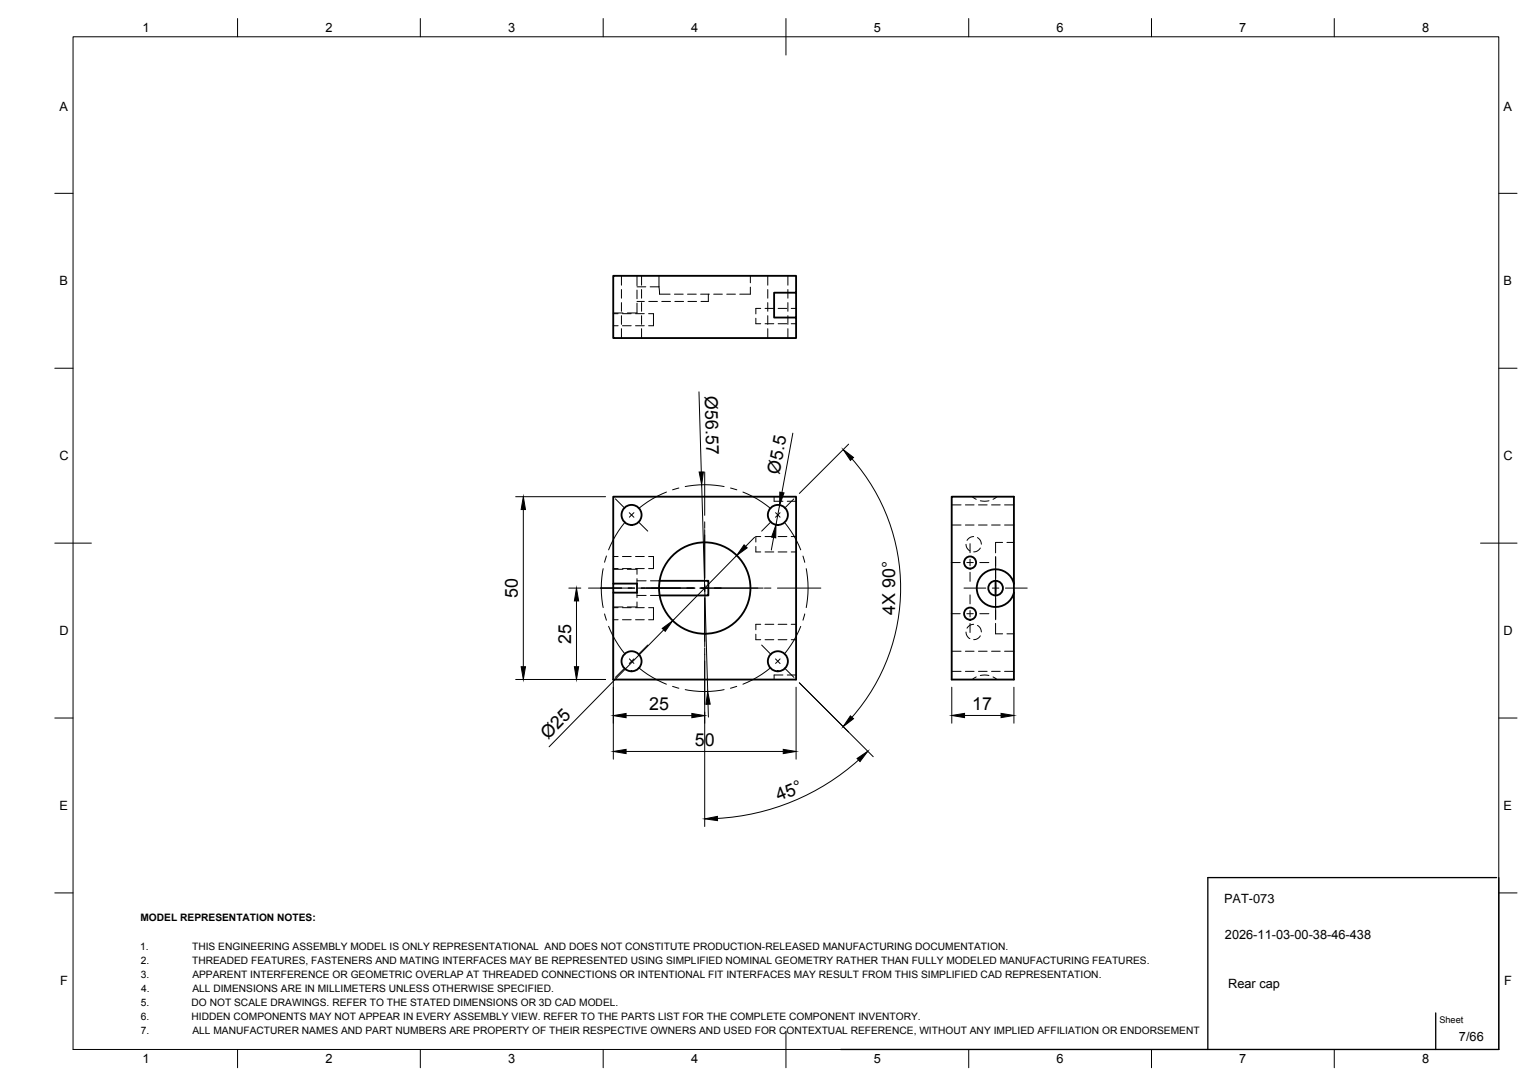
ISO-10303-21;
HEADER;
/* Generated by software containing ST-Developer
 * from STEP Tools, Inc. (www.steptools.com) 
 */

FILE_DESCRIPTION(
/* description */ ('Manual piston pump'),
/* implementation_level */ '2;1');

FILE_NAME(
/* name */ 'Rear cap.step',
/* time_stamp */ '2026-11-02T16:54:23-08:00',
/* author */ (''),
/* organization */ (''),
/* preprocessor_version */ 'ST-DEVELOPER v20.2',
/* originating_system */ 'Autodesk Translation Framework v15.17.0.0',
/* authorisation */ '');

FILE_SCHEMA (('AUTOMOTIVE_DESIGN { 1 0 10303 214 3 1 1 }'));
ENDSEC;

DATA;
#10=MECHANICAL_DESIGN_GEOMETRIC_PRESENTATION_REPRESENTATION('',(#690),#19043);
#564=SHAPE_REPRESENTATION_RELATIONSHIP('SRR','None',#19310,#627);
#627=ADVANCED_BREP_SHAPE_REPRESENTATION('',(#762),#18977);
#690=STYLED_ITEM('',(#19661),#762);
#762=MANIFOLD_SOLID_BREP('Body1',#9474);
#850=FACE_BOUND('',#1945,.T.);
#851=FACE_BOUND('',#1948,.T.);
#852=FACE_BOUND('',#1949,.T.);
#853=FACE_BOUND('',#1950,.T.);
#854=FACE_BOUND('',#1951,.T.);
#855=FACE_BOUND('',#1952,.T.);
#856=FACE_BOUND('',#1959,.T.);
#857=FACE_BOUND('',#1960,.T.);
#858=FACE_BOUND('',#1961,.T.);
#859=FACE_BOUND('',#1962,.T.);
#860=FACE_BOUND('',#1965,.T.);
#861=FACE_BOUND('',#1966,.T.);
#862=FACE_BOUND('',#1968,.T.);
#863=FACE_BOUND('',#1969,.T.);
#1050=B_SPLINE_CURVE_WITH_KNOTS('',3,(#14902,#14903,#14904,#14905,#14906,
#14907,#14908,#14909,#14910,#14911,#14912,#14913,#14914,#14915,#14916,#14917,
#14918,#14919),.UNSPECIFIED.,.F.,.F.,(4,2,2,2,2,2,2,2,4),(-0.603815071984235,
-0.528337333647547,-0.45285959531086,-0.377383565651489,-0.301907535992118,
-0.226431506332746,-0.150955476673375,-0.0754777383366876,0.),
 .UNSPECIFIED.);
#1109=CYLINDRICAL_SURFACE('',#10323,0.165);
#1110=CYLINDRICAL_SURFACE('',#10327,0.165);
#1111=CYLINDRICAL_SURFACE('',#10333,0.525);
#1112=CYLINDRICAL_SURFACE('',#10335,0.525);
#1113=CYLINDRICAL_SURFACE('',#10340,0.21);
#1114=CYLINDRICAL_SURFACE('',#10344,0.21);
#1115=CYLINDRICAL_SURFACE('',#10350,0.2);
#1116=CYLINDRICAL_SURFACE('',#10357,0.515);
#1117=CYLINDRICAL_SURFACE('',#10365,0.275);
#1118=CYLINDRICAL_SURFACE('',#10367,0.275);
#1119=CYLINDRICAL_SURFACE('',#10369,0.275);
#1120=CYLINDRICAL_SURFACE('',#10371,0.275);
#1121=CYLINDRICAL_SURFACE('',#10373,1.25);
#1330=FACE_OUTER_BOUND('',#1928,.T.);
#1331=FACE_OUTER_BOUND('',#1929,.T.);
#1332=FACE_OUTER_BOUND('',#1930,.T.);
#1333=FACE_OUTER_BOUND('',#1931,.T.);
#1334=FACE_OUTER_BOUND('',#1932,.T.);
#1335=FACE_OUTER_BOUND('',#1933,.T.);
#1336=FACE_OUTER_BOUND('',#1934,.T.);
#1337=FACE_OUTER_BOUND('',#1935,.T.);
#1338=FACE_OUTER_BOUND('',#1936,.T.);
#1339=FACE_OUTER_BOUND('',#1937,.T.);
#1340=FACE_OUTER_BOUND('',#1938,.T.);
#1341=FACE_OUTER_BOUND('',#1939,.T.);
#1342=FACE_OUTER_BOUND('',#1940,.T.);
#1343=FACE_OUTER_BOUND('',#1941,.T.);
#1344=FACE_OUTER_BOUND('',#1942,.T.);
#1345=FACE_OUTER_BOUND('',#1943,.T.);
#1346=FACE_OUTER_BOUND('',#1944,.T.);
#1347=FACE_OUTER_BOUND('',#1946,.T.);
#1348=FACE_OUTER_BOUND('',#1947,.T.);
#1349=FACE_OUTER_BOUND('',#1953,.T.);
#1350=FACE_OUTER_BOUND('',#1954,.T.);
#1351=FACE_OUTER_BOUND('',#1955,.T.);
#1352=FACE_OUTER_BOUND('',#1956,.T.);
#1353=FACE_OUTER_BOUND('',#1957,.T.);
#1354=FACE_OUTER_BOUND('',#1958,.T.);
#1355=FACE_OUTER_BOUND('',#1963,.T.);
#1356=FACE_OUTER_BOUND('',#1964,.T.);
#1357=FACE_OUTER_BOUND('',#1967,.T.);
#1928=EDGE_LOOP('',(#6457,#6458,#6459,#6460));
#1929=EDGE_LOOP('',(#6461));
#1930=EDGE_LOOP('',(#6462,#6463,#6464,#6465));
#1931=EDGE_LOOP('',(#6466));
#1932=EDGE_LOOP('',(#6467,#6468));
#1933=EDGE_LOOP('',(#6469,#6470,#6471,#6472));
#1934=EDGE_LOOP('',(#6473,#6474,#6475,#6476));
#1935=EDGE_LOOP('',(#6477,#6478));
#1936=EDGE_LOOP('',(#6479,#6480,#6481,#6482,#6483,#6484,#6485,#6486));
#1937=EDGE_LOOP('',(#6487,#6488,#6489,#6490));
#1938=EDGE_LOOP('',(#6491));
#1939=EDGE_LOOP('',(#6492,#6493,#6494,#6495));
#1940=EDGE_LOOP('',(#6496));
#1941=EDGE_LOOP('',(#6497,#6498));
#1942=EDGE_LOOP('',(#6499,#6500,#6501,#6502,#6503,#6504,#6505));
#1943=EDGE_LOOP('',(#6506,#6507,#6508,#6509,#6510));
#1944=EDGE_LOOP('',(#6511,#6512));
#1945=EDGE_LOOP('',(#6513));
#1946=EDGE_LOOP('',(#6514,#6515,#6516,#6517));
#1947=EDGE_LOOP('',(#6518,#6519,#6520,#6521,#6522,#6523,#6524,#6525));
#1948=EDGE_LOOP('',(#6526));
#1949=EDGE_LOOP('',(#6527));
#1950=EDGE_LOOP('',(#6528));
#1951=EDGE_LOOP('',(#6529));
#1952=EDGE_LOOP('',(#6530));
#1953=EDGE_LOOP('',(#6531,#6532,#6533,#6534));
#1954=EDGE_LOOP('',(#6535,#6536,#6537,#6538));
#1955=EDGE_LOOP('',(#6539,#6540,#6541,#6542));
#1956=EDGE_LOOP('',(#6543,#6544,#6545,#6546));
#1957=EDGE_LOOP('',(#6547,#6548,#6549,#6550,#6551,#6552));
#1958=EDGE_LOOP('',(#6553,#6554,#6555,#6556));
#1959=EDGE_LOOP('',(#6557));
#1960=EDGE_LOOP('',(#6558));
#1961=EDGE_LOOP('',(#6559));
#1962=EDGE_LOOP('',(#6560));
#1963=EDGE_LOOP('',(#6561,#6562,#6563,#6564,#6565,#6566,#6567,#6568));
#1964=EDGE_LOOP('',(#6569,#6570,#6571,#6572,#6573,#6574));
#1965=EDGE_LOOP('',(#6575));
#1966=EDGE_LOOP('',(#6576));
#1967=EDGE_LOOP('',(#6577,#6578,#6579,#6580,#6581,#6582,#6583,#6584));
#1968=EDGE_LOOP('',(#6585));
#1969=EDGE_LOOP('',(#6586));
#2700=CIRCLE('',#10324,0.165);
#2701=CIRCLE('',#10325,0.165);
#2702=CIRCLE('',#10328,0.165);
#2703=CIRCLE('',#10329,0.165);
#2704=CIRCLE('',#10332,0.525);
#2705=CIRCLE('',#10334,0.525);
#2706=CIRCLE('',#10336,0.525);
#2707=CIRCLE('',#10337,0.525);
#2708=CIRCLE('',#10341,0.21);
#2709=CIRCLE('',#10342,0.21);
#2710=CIRCLE('',#10345,0.21);
#2711=CIRCLE('',#10346,0.21);
#2712=CIRCLE('',#10349,0.2);
#2713=CIRCLE('',#10351,0.2);
#2714=CIRCLE('',#10353,1.25);
#2715=CIRCLE('',#10354,1.25);
#2716=CIRCLE('',#10356,0.515);
#2717=CIRCLE('',#10358,0.515);
#2718=CIRCLE('',#10360,0.275);
#2719=CIRCLE('',#10361,0.275);
#2720=CIRCLE('',#10362,0.275);
#2721=CIRCLE('',#10363,0.275);
#2722=CIRCLE('',#10364,1.25);
#2723=CIRCLE('',#10366,0.275);
#2724=CIRCLE('',#10368,0.275);
#2725=CIRCLE('',#10370,0.275);
#2726=CIRCLE('',#10372,0.275);
#3200=LINE('',#14837,#3804);
#3201=LINE('',#14844,#3805);
#3202=LINE('',#14850,#3806);
#3203=LINE('',#14854,#3807);
#3204=LINE('',#14857,#3808);
#3205=LINE('',#14861,#3809);
#3206=LINE('',#14865,#3810);
#3207=LINE('',#14868,#3811);
#3208=LINE('',#14871,#3812);
#3209=LINE('',#14873,#3813);
#3210=LINE('',#14875,#3814);
#3211=LINE('',#14877,#3815);
#3212=LINE('',#14878,#3816);
#3213=LINE('',#14883,#3817);
#3214=LINE('',#14890,#3818);
#3215=LINE('',#14896,#3819);
#3216=LINE('',#14900,#3820);
#3217=LINE('',#14921,#3821);
#3218=LINE('',#14923,#3822);
#3219=LINE('',#14931,#3823);
#3220=LINE('',#14935,#3824);
#3221=LINE('',#14938,#3825);
#3222=LINE('',#14940,#3826);
#3223=LINE('',#14942,#3827);
#3224=LINE('',#14944,#3828);
#3225=LINE('',#14945,#3829);
#3226=LINE('',#14958,#3830);
#3227=LINE('',#14962,#3831);
#3228=LINE('',#14966,#3832);
#3229=LINE('',#14970,#3833);
#3230=LINE('',#14973,#3834);
#3231=LINE('',#14976,#3835);
#3232=LINE('',#14978,#3836);
#3233=LINE('',#14979,#3837);
#3234=LINE('',#14981,#3838);
#3235=LINE('',#14982,#3839);
#3236=LINE('',#14983,#3840);
#3804=VECTOR('',#11712,0.165);
#3805=VECTOR('',#11721,0.165);
#3806=VECTOR('',#11728,1.);
#3807=VECTOR('',#11733,1.);
#3808=VECTOR('',#11736,1.);
#3809=VECTOR('',#11739,1.);
#3810=VECTOR('',#11742,1.);
#3811=VECTOR('',#11747,1.);
#3812=VECTOR('',#11750,1.);
#3813=VECTOR('',#11751,1.);
#3814=VECTOR('',#11752,1.);
#3815=VECTOR('',#11753,1.);
#3816=VECTOR('',#11754,1.);
#3817=VECTOR('',#11759,0.21);
#3818=VECTOR('',#11768,0.21);
#3819=VECTOR('',#11775,1.);
#3820=VECTOR('',#11780,1.);
#3821=VECTOR('',#11781,0.2);
#3822=VECTOR('',#11784,1.);
#3823=VECTOR('',#11793,1.);
#3824=VECTOR('',#11798,1.);
#3825=VECTOR('',#11801,1.);
#3826=VECTOR('',#11804,1.);
#3827=VECTOR('',#11805,1.);
#3828=VECTOR('',#11806,1.);
#3829=VECTOR('',#11807,1.);
#3830=VECTOR('',#11820,0.275);
#3831=VECTOR('',#11825,0.275);
#3832=VECTOR('',#11830,0.275);
#3833=VECTOR('',#11835,0.275);
#3834=VECTOR('',#11840,1.25);
#3835=VECTOR('',#11843,1.);
#3836=VECTOR('',#11844,1.);
#3837=VECTOR('',#11845,1.);
#3838=VECTOR('',#11848,1.);
#3839=VECTOR('',#11849,1.);
#3840=VECTOR('',#11850,1.);
#4416=VERTEX_POINT('',#14834);
#4417=VERTEX_POINT('',#14836);
#4418=VERTEX_POINT('',#14841);
#4419=VERTEX_POINT('',#14843);
#4420=VERTEX_POINT('',#14848);
#4421=VERTEX_POINT('',#14849);
#4422=VERTEX_POINT('',#14853);
#4423=VERTEX_POINT('',#14855);
#4424=VERTEX_POINT('',#14859);
#4425=VERTEX_POINT('',#14860);
#4426=VERTEX_POINT('',#14862);
#4427=VERTEX_POINT('',#14864);
#4428=VERTEX_POINT('',#14870);
#4429=VERTEX_POINT('',#14872);
#4430=VERTEX_POINT('',#14874);
#4431=VERTEX_POINT('',#14876);
#4432=VERTEX_POINT('',#14880);
#4433=VERTEX_POINT('',#14882);
#4434=VERTEX_POINT('',#14887);
#4435=VERTEX_POINT('',#14889);
#4436=VERTEX_POINT('',#14894);
#4437=VERTEX_POINT('',#14895);
#4438=VERTEX_POINT('',#14899);
#4439=VERTEX_POINT('',#14901);
#4440=VERTEX_POINT('',#14920);
#4441=VERTEX_POINT('',#14925);
#4442=VERTEX_POINT('',#14929);
#4443=VERTEX_POINT('',#14930);
#4444=VERTEX_POINT('',#14934);
#4445=VERTEX_POINT('',#14936);
#4446=VERTEX_POINT('',#14941);
#4447=VERTEX_POINT('',#14943);
#4448=VERTEX_POINT('',#14946);
#4449=VERTEX_POINT('',#14948);
#4450=VERTEX_POINT('',#14950);
#4451=VERTEX_POINT('',#14952);
#4452=VERTEX_POINT('',#14954);
#4453=VERTEX_POINT('',#14957);
#4454=VERTEX_POINT('',#14961);
#4455=VERTEX_POINT('',#14965);
#4456=VERTEX_POINT('',#14969);
#4457=VERTEX_POINT('',#14975);
#4458=VERTEX_POINT('',#14977);
#5215=EDGE_CURVE('',#4416,#4416,#2700,.T.);
#5216=EDGE_CURVE('',#4416,#4417,#3200,.T.);
#5217=EDGE_CURVE('',#4417,#4417,#2701,.T.);
#5218=EDGE_CURVE('',#4418,#4418,#2702,.T.);
#5219=EDGE_CURVE('',#4418,#4419,#3201,.T.);
#5220=EDGE_CURVE('',#4419,#4419,#2703,.T.);
#5221=EDGE_CURVE('',#4420,#4421,#3202,.T.);
#5222=EDGE_CURVE('',#4421,#4420,#2704,.T.);
#5223=EDGE_CURVE('',#4422,#4420,#3203,.T.);
#5224=EDGE_CURVE('',#4423,#4422,#2705,.T.);
#5225=EDGE_CURVE('',#4421,#4423,#3204,.T.);
#5226=EDGE_CURVE('',#4424,#4425,#3205,.T.);
#5227=EDGE_CURVE('',#4424,#4426,#2706,.T.);
#5228=EDGE_CURVE('',#4427,#4426,#3206,.T.);
#5229=EDGE_CURVE('',#4425,#4427,#2707,.T.);
#5230=EDGE_CURVE('',#4426,#4424,#3207,.T.);
#5231=EDGE_CURVE('',#4423,#4428,#3208,.T.);
#5232=EDGE_CURVE('',#4428,#4429,#3209,.T.);
#5233=EDGE_CURVE('',#4430,#4429,#3210,.T.);
#5234=EDGE_CURVE('',#4431,#4430,#3211,.T.);
#5235=EDGE_CURVE('',#4431,#4422,#3212,.T.);
#5236=EDGE_CURVE('',#4432,#4432,#2708,.T.);
#5237=EDGE_CURVE('',#4432,#4433,#3213,.T.);
#5238=EDGE_CURVE('',#4433,#4433,#2709,.T.);
#5239=EDGE_CURVE('',#4434,#4434,#2710,.T.);
#5240=EDGE_CURVE('',#4434,#4435,#3214,.T.);
#5241=EDGE_CURVE('',#4435,#4435,#2711,.T.);
#5242=EDGE_CURVE('',#4436,#4437,#3215,.T.);
#5243=EDGE_CURVE('',#4436,#4437,#2712,.T.);
#5244=EDGE_CURVE('',#4438,#4436,#3216,.T.);
#5245=EDGE_CURVE('',#4439,#4438,#1050,.T.);
#5246=EDGE_CURVE('',#4439,#4440,#3217,.T.);
#5247=EDGE_CURVE('',#4440,#4440,#2713,.T.);
#5248=EDGE_CURVE('',#4437,#4439,#3218,.T.);
#5249=EDGE_CURVE('',#4441,#4439,#2714,.T.);
#5250=EDGE_CURVE('',#4438,#4441,#2715,.T.);
#5251=EDGE_CURVE('',#4442,#4443,#3219,.T.);
#5252=EDGE_CURVE('',#4442,#4443,#2716,.T.);
#5253=EDGE_CURVE('',#4444,#4442,#3220,.T.);
#5254=EDGE_CURVE('',#4445,#4444,#2717,.T.);
#5255=EDGE_CURVE('',#4443,#4445,#3221,.T.);
#5256=EDGE_CURVE('',#4429,#4445,#3222,.T.);
#5257=EDGE_CURVE('',#4428,#4446,#3223,.T.);
#5258=EDGE_CURVE('',#4446,#4447,#3224,.T.);
#5259=EDGE_CURVE('',#4444,#4447,#3225,.T.);
#5260=EDGE_CURVE('',#4448,#4448,#2718,.T.);
#5261=EDGE_CURVE('',#4449,#4449,#2719,.T.);
#5262=EDGE_CURVE('',#4450,#4450,#2720,.T.);
#5263=EDGE_CURVE('',#4451,#4451,#2721,.T.);
#5264=EDGE_CURVE('',#4452,#4452,#2722,.T.);
#5265=EDGE_CURVE('',#4448,#4453,#3226,.T.);
#5266=EDGE_CURVE('',#4453,#4453,#2723,.T.);
#5267=EDGE_CURVE('',#4449,#4454,#3227,.T.);
#5268=EDGE_CURVE('',#4454,#4454,#2724,.T.);
#5269=EDGE_CURVE('',#4450,#4455,#3228,.T.);
#5270=EDGE_CURVE('',#4455,#4455,#2725,.T.);
#5271=EDGE_CURVE('',#4451,#4456,#3229,.T.);
#5272=EDGE_CURVE('',#4456,#4456,#2726,.T.);
#5273=EDGE_CURVE('',#4452,#4441,#3230,.T.);
#5274=EDGE_CURVE('',#4457,#4431,#3231,.T.);
#5275=EDGE_CURVE('',#4458,#4430,#3232,.T.);
#5276=EDGE_CURVE('',#4457,#4458,#3233,.T.);
#5277=EDGE_CURVE('',#4425,#4457,#3234,.T.);
#5278=EDGE_CURVE('',#4447,#4458,#3235,.T.);
#5279=EDGE_CURVE('',#4446,#4427,#3236,.T.);
#6457=ORIENTED_EDGE('',*,*,#5215,.F.);
#6458=ORIENTED_EDGE('',*,*,#5216,.T.);
#6459=ORIENTED_EDGE('',*,*,#5217,.F.);
#6460=ORIENTED_EDGE('',*,*,#5216,.F.);
#6461=ORIENTED_EDGE('',*,*,#5215,.T.);
#6462=ORIENTED_EDGE('',*,*,#5218,.F.);
#6463=ORIENTED_EDGE('',*,*,#5219,.T.);
#6464=ORIENTED_EDGE('',*,*,#5220,.F.);
#6465=ORIENTED_EDGE('',*,*,#5219,.F.);
#6466=ORIENTED_EDGE('',*,*,#5218,.T.);
#6467=ORIENTED_EDGE('',*,*,#5221,.F.);
#6468=ORIENTED_EDGE('',*,*,#5222,.F.);
#6469=ORIENTED_EDGE('',*,*,#5223,.F.);
#6470=ORIENTED_EDGE('',*,*,#5224,.F.);
#6471=ORIENTED_EDGE('',*,*,#5225,.F.);
#6472=ORIENTED_EDGE('',*,*,#5222,.T.);
#6473=ORIENTED_EDGE('',*,*,#5226,.F.);
#6474=ORIENTED_EDGE('',*,*,#5227,.T.);
#6475=ORIENTED_EDGE('',*,*,#5228,.F.);
#6476=ORIENTED_EDGE('',*,*,#5229,.F.);
#6477=ORIENTED_EDGE('',*,*,#5230,.F.);
#6478=ORIENTED_EDGE('',*,*,#5227,.F.);
#6479=ORIENTED_EDGE('',*,*,#5223,.T.);
#6480=ORIENTED_EDGE('',*,*,#5221,.T.);
#6481=ORIENTED_EDGE('',*,*,#5225,.T.);
#6482=ORIENTED_EDGE('',*,*,#5231,.T.);
#6483=ORIENTED_EDGE('',*,*,#5232,.T.);
#6484=ORIENTED_EDGE('',*,*,#5233,.F.);
#6485=ORIENTED_EDGE('',*,*,#5234,.F.);
#6486=ORIENTED_EDGE('',*,*,#5235,.T.);
#6487=ORIENTED_EDGE('',*,*,#5236,.F.);
#6488=ORIENTED_EDGE('',*,*,#5237,.T.);
#6489=ORIENTED_EDGE('',*,*,#5238,.T.);
#6490=ORIENTED_EDGE('',*,*,#5237,.F.);
#6491=ORIENTED_EDGE('',*,*,#5238,.F.);
#6492=ORIENTED_EDGE('',*,*,#5239,.F.);
#6493=ORIENTED_EDGE('',*,*,#5240,.T.);
#6494=ORIENTED_EDGE('',*,*,#5241,.T.);
#6495=ORIENTED_EDGE('',*,*,#5240,.F.);
#6496=ORIENTED_EDGE('',*,*,#5241,.F.);
#6497=ORIENTED_EDGE('',*,*,#5242,.F.);
#6498=ORIENTED_EDGE('',*,*,#5243,.T.);
#6499=ORIENTED_EDGE('',*,*,#5244,.F.);
#6500=ORIENTED_EDGE('',*,*,#5245,.F.);
#6501=ORIENTED_EDGE('',*,*,#5246,.T.);
#6502=ORIENTED_EDGE('',*,*,#5247,.F.);
#6503=ORIENTED_EDGE('',*,*,#5246,.F.);
#6504=ORIENTED_EDGE('',*,*,#5248,.F.);
#6505=ORIENTED_EDGE('',*,*,#5243,.F.);
#6506=ORIENTED_EDGE('',*,*,#5244,.T.);
#6507=ORIENTED_EDGE('',*,*,#5242,.T.);
#6508=ORIENTED_EDGE('',*,*,#5248,.T.);
#6509=ORIENTED_EDGE('',*,*,#5249,.F.);
#6510=ORIENTED_EDGE('',*,*,#5250,.F.);
#6511=ORIENTED_EDGE('',*,*,#5251,.F.);
#6512=ORIENTED_EDGE('',*,*,#5252,.T.);
#6513=ORIENTED_EDGE('',*,*,#5247,.T.);
#6514=ORIENTED_EDGE('',*,*,#5253,.F.);
#6515=ORIENTED_EDGE('',*,*,#5254,.F.);
#6516=ORIENTED_EDGE('',*,*,#5255,.F.);
#6517=ORIENTED_EDGE('',*,*,#5252,.F.);
#6518=ORIENTED_EDGE('',*,*,#5253,.T.);
#6519=ORIENTED_EDGE('',*,*,#5251,.T.);
#6520=ORIENTED_EDGE('',*,*,#5255,.T.);
#6521=ORIENTED_EDGE('',*,*,#5256,.F.);
#6522=ORIENTED_EDGE('',*,*,#5232,.F.);
#6523=ORIENTED_EDGE('',*,*,#5257,.T.);
#6524=ORIENTED_EDGE('',*,*,#5258,.T.);
#6525=ORIENTED_EDGE('',*,*,#5259,.F.);
#6526=ORIENTED_EDGE('',*,*,#5260,.T.);
#6527=ORIENTED_EDGE('',*,*,#5261,.T.);
#6528=ORIENTED_EDGE('',*,*,#5262,.T.);
#6529=ORIENTED_EDGE('',*,*,#5263,.T.);
#6530=ORIENTED_EDGE('',*,*,#5264,.T.);
#6531=ORIENTED_EDGE('',*,*,#5260,.F.);
#6532=ORIENTED_EDGE('',*,*,#5265,.T.);
#6533=ORIENTED_EDGE('',*,*,#5266,.F.);
#6534=ORIENTED_EDGE('',*,*,#5265,.F.);
#6535=ORIENTED_EDGE('',*,*,#5261,.F.);
#6536=ORIENTED_EDGE('',*,*,#5267,.T.);
#6537=ORIENTED_EDGE('',*,*,#5268,.F.);
#6538=ORIENTED_EDGE('',*,*,#5267,.F.);
#6539=ORIENTED_EDGE('',*,*,#5262,.F.);
#6540=ORIENTED_EDGE('',*,*,#5269,.T.);
#6541=ORIENTED_EDGE('',*,*,#5270,.F.);
#6542=ORIENTED_EDGE('',*,*,#5269,.F.);
#6543=ORIENTED_EDGE('',*,*,#5263,.F.);
#6544=ORIENTED_EDGE('',*,*,#5271,.T.);
#6545=ORIENTED_EDGE('',*,*,#5272,.F.);
#6546=ORIENTED_EDGE('',*,*,#5271,.F.);
#6547=ORIENTED_EDGE('',*,*,#5264,.F.);
#6548=ORIENTED_EDGE('',*,*,#5273,.T.);
#6549=ORIENTED_EDGE('',*,*,#5249,.T.);
#6550=ORIENTED_EDGE('',*,*,#5245,.T.);
#6551=ORIENTED_EDGE('',*,*,#5250,.T.);
#6552=ORIENTED_EDGE('',*,*,#5273,.F.);
#6553=ORIENTED_EDGE('',*,*,#5274,.T.);
#6554=ORIENTED_EDGE('',*,*,#5234,.T.);
#6555=ORIENTED_EDGE('',*,*,#5275,.F.);
#6556=ORIENTED_EDGE('',*,*,#5276,.F.);
#6557=ORIENTED_EDGE('',*,*,#5266,.T.);
#6558=ORIENTED_EDGE('',*,*,#5268,.T.);
#6559=ORIENTED_EDGE('',*,*,#5270,.T.);
#6560=ORIENTED_EDGE('',*,*,#5272,.T.);
#6561=ORIENTED_EDGE('',*,*,#5226,.T.);
#6562=ORIENTED_EDGE('',*,*,#5277,.T.);
#6563=ORIENTED_EDGE('',*,*,#5276,.T.);
#6564=ORIENTED_EDGE('',*,*,#5278,.F.);
#6565=ORIENTED_EDGE('',*,*,#5258,.F.);
#6566=ORIENTED_EDGE('',*,*,#5279,.T.);
#6567=ORIENTED_EDGE('',*,*,#5228,.T.);
#6568=ORIENTED_EDGE('',*,*,#5230,.T.);
#6569=ORIENTED_EDGE('',*,*,#5254,.T.);
#6570=ORIENTED_EDGE('',*,*,#5259,.T.);
#6571=ORIENTED_EDGE('',*,*,#5278,.T.);
#6572=ORIENTED_EDGE('',*,*,#5275,.T.);
#6573=ORIENTED_EDGE('',*,*,#5233,.T.);
#6574=ORIENTED_EDGE('',*,*,#5256,.T.);
#6575=ORIENTED_EDGE('',*,*,#5217,.T.);
#6576=ORIENTED_EDGE('',*,*,#5220,.T.);
#6577=ORIENTED_EDGE('',*,*,#5224,.T.);
#6578=ORIENTED_EDGE('',*,*,#5235,.F.);
#6579=ORIENTED_EDGE('',*,*,#5274,.F.);
#6580=ORIENTED_EDGE('',*,*,#5277,.F.);
#6581=ORIENTED_EDGE('',*,*,#5229,.T.);
#6582=ORIENTED_EDGE('',*,*,#5279,.F.);
#6583=ORIENTED_EDGE('',*,*,#5257,.F.);
#6584=ORIENTED_EDGE('',*,*,#5231,.F.);
#6585=ORIENTED_EDGE('',*,*,#5236,.T.);
#6586=ORIENTED_EDGE('',*,*,#5239,.T.);
#8593=PLANE('',#10326);
#8594=PLANE('',#10330);
#8595=PLANE('',#10331);
#8596=PLANE('',#10338);
#8597=PLANE('',#10339);
#8598=PLANE('',#10343);
#8599=PLANE('',#10347);
#8600=PLANE('',#10348);
#8601=PLANE('',#10352);
#8602=PLANE('',#10355);
#8603=PLANE('',#10359);
#8604=PLANE('',#10374);
#8605=PLANE('',#10375);
#8606=PLANE('',#10376);
#8607=PLANE('',#10377);
#8935=ADVANCED_FACE('',(#1330),#1109,.F.);
#8936=ADVANCED_FACE('',(#1331),#8593,.T.);
#8937=ADVANCED_FACE('',(#1332),#1110,.F.);
#8938=ADVANCED_FACE('',(#1333),#8594,.T.);
#8939=ADVANCED_FACE('',(#1334),#8595,.F.);
#8940=ADVANCED_FACE('',(#1335),#1111,.F.);
#8941=ADVANCED_FACE('',(#1336),#1112,.F.);
#8942=ADVANCED_FACE('',(#1337),#8596,.F.);
#8943=ADVANCED_FACE('',(#1338),#8597,.T.);
#8944=ADVANCED_FACE('',(#1339),#1113,.F.);
#8945=ADVANCED_FACE('',(#1340),#8598,.F.);
#8946=ADVANCED_FACE('',(#1341),#1114,.F.);
#8947=ADVANCED_FACE('',(#1342),#8599,.F.);
#8948=ADVANCED_FACE('',(#1343),#8600,.T.);
#8949=ADVANCED_FACE('',(#1344),#1115,.F.);
#8950=ADVANCED_FACE('',(#1345),#8601,.F.);
#8951=ADVANCED_FACE('',(#1346,#850),#8602,.T.);
#8952=ADVANCED_FACE('',(#1347),#1116,.F.);
#8953=ADVANCED_FACE('',(#1348,#851,#852,#853,#854,#855),#8603,.T.);
#8954=ADVANCED_FACE('',(#1349),#1117,.F.);
#8955=ADVANCED_FACE('',(#1350),#1118,.F.);
#8956=ADVANCED_FACE('',(#1351),#1119,.F.);
#8957=ADVANCED_FACE('',(#1352),#1120,.F.);
#8958=ADVANCED_FACE('',(#1353),#1121,.F.);
#8959=ADVANCED_FACE('',(#1354,#856,#857,#858,#859),#8604,.T.);
#8960=ADVANCED_FACE('',(#1355),#8605,.T.);
#8961=ADVANCED_FACE('',(#1356,#860,#861),#8606,.T.);
#8962=ADVANCED_FACE('',(#1357,#862,#863),#8607,.F.);
#9474=CLOSED_SHELL('',(#8935,#8936,#8937,#8938,#8939,#8940,#8941,#8942,
#8943,#8944,#8945,#8946,#8947,#8948,#8949,#8950,#8951,#8952,#8953,#8954,
#8955,#8956,#8957,#8958,#8959,#8960,#8961,#8962));
#10322=AXIS2_PLACEMENT_3D('',#14832,#11706,#11707);
#10323=AXIS2_PLACEMENT_3D('',#14833,#11708,#11709);
#10324=AXIS2_PLACEMENT_3D('',#14835,#11710,#11711);
#10325=AXIS2_PLACEMENT_3D('',#14838,#11713,#11714);
#10326=AXIS2_PLACEMENT_3D('',#14839,#11715,#11716);
#10327=AXIS2_PLACEMENT_3D('',#14840,#11717,#11718);
#10328=AXIS2_PLACEMENT_3D('',#14842,#11719,#11720);
#10329=AXIS2_PLACEMENT_3D('',#14845,#11722,#11723);
#10330=AXIS2_PLACEMENT_3D('',#14846,#11724,#11725);
#10331=AXIS2_PLACEMENT_3D('',#14847,#11726,#11727);
#10332=AXIS2_PLACEMENT_3D('',#14851,#11729,#11730);
#10333=AXIS2_PLACEMENT_3D('',#14852,#11731,#11732);
#10334=AXIS2_PLACEMENT_3D('',#14856,#11734,#11735);
#10335=AXIS2_PLACEMENT_3D('',#14858,#11737,#11738);
#10336=AXIS2_PLACEMENT_3D('',#14863,#11740,#11741);
#10337=AXIS2_PLACEMENT_3D('',#14866,#11743,#11744);
#10338=AXIS2_PLACEMENT_3D('',#14867,#11745,#11746);
#10339=AXIS2_PLACEMENT_3D('',#14869,#11748,#11749);
#10340=AXIS2_PLACEMENT_3D('',#14879,#11755,#11756);
#10341=AXIS2_PLACEMENT_3D('',#14881,#11757,#11758);
#10342=AXIS2_PLACEMENT_3D('',#14884,#11760,#11761);
#10343=AXIS2_PLACEMENT_3D('',#14885,#11762,#11763);
#10344=AXIS2_PLACEMENT_3D('',#14886,#11764,#11765);
#10345=AXIS2_PLACEMENT_3D('',#14888,#11766,#11767);
#10346=AXIS2_PLACEMENT_3D('',#14891,#11769,#11770);
#10347=AXIS2_PLACEMENT_3D('',#14892,#11771,#11772);
#10348=AXIS2_PLACEMENT_3D('',#14893,#11773,#11774);
#10349=AXIS2_PLACEMENT_3D('',#14897,#11776,#11777);
#10350=AXIS2_PLACEMENT_3D('',#14898,#11778,#11779);
#10351=AXIS2_PLACEMENT_3D('',#14922,#11782,#11783);
#10352=AXIS2_PLACEMENT_3D('',#14924,#11785,#11786);
#10353=AXIS2_PLACEMENT_3D('',#14926,#11787,#11788);
#10354=AXIS2_PLACEMENT_3D('',#14927,#11789,#11790);
#10355=AXIS2_PLACEMENT_3D('',#14928,#11791,#11792);
#10356=AXIS2_PLACEMENT_3D('',#14932,#11794,#11795);
#10357=AXIS2_PLACEMENT_3D('',#14933,#11796,#11797);
#10358=AXIS2_PLACEMENT_3D('',#14937,#11799,#11800);
#10359=AXIS2_PLACEMENT_3D('',#14939,#11802,#11803);
#10360=AXIS2_PLACEMENT_3D('',#14947,#11808,#11809);
#10361=AXIS2_PLACEMENT_3D('',#14949,#11810,#11811);
#10362=AXIS2_PLACEMENT_3D('',#14951,#11812,#11813);
#10363=AXIS2_PLACEMENT_3D('',#14953,#11814,#11815);
#10364=AXIS2_PLACEMENT_3D('',#14955,#11816,#11817);
#10365=AXIS2_PLACEMENT_3D('',#14956,#11818,#11819);
#10366=AXIS2_PLACEMENT_3D('',#14959,#11821,#11822);
#10367=AXIS2_PLACEMENT_3D('',#14960,#11823,#11824);
#10368=AXIS2_PLACEMENT_3D('',#14963,#11826,#11827);
#10369=AXIS2_PLACEMENT_3D('',#14964,#11828,#11829);
#10370=AXIS2_PLACEMENT_3D('',#14967,#11831,#11832);
#10371=AXIS2_PLACEMENT_3D('',#14968,#11833,#11834);
#10372=AXIS2_PLACEMENT_3D('',#14971,#11836,#11837);
#10373=AXIS2_PLACEMENT_3D('',#14972,#11838,#11839);
#10374=AXIS2_PLACEMENT_3D('',#14974,#11841,#11842);
#10375=AXIS2_PLACEMENT_3D('',#14980,#11846,#11847);
#10376=AXIS2_PLACEMENT_3D('',#14984,#11851,#11852);
#10377=AXIS2_PLACEMENT_3D('',#14985,#11853,#11854);
#11706=DIRECTION('axis',(0.,0.,1.));
#11707=DIRECTION('refdir',(1.,0.,0.));
#11708=DIRECTION('center_axis',(0.,0.,1.));
#11709=DIRECTION('ref_axis',(1.,0.,0.));
#11710=DIRECTION('center_axis',(0.,0.,1.));
#11711=DIRECTION('ref_axis',(1.,0.,0.));
#11712=DIRECTION('',(0.,0.,1.));
#11713=DIRECTION('center_axis',(0.,0.,-1.));
#11714=DIRECTION('ref_axis',(1.,0.,0.));
#11715=DIRECTION('center_axis',(0.,0.,1.));
#11716=DIRECTION('ref_axis',(1.,0.,0.));
#11717=DIRECTION('center_axis',(0.,0.,1.));
#11718=DIRECTION('ref_axis',(1.,0.,0.));
#11719=DIRECTION('center_axis',(0.,0.,1.));
#11720=DIRECTION('ref_axis',(1.,0.,0.));
#11721=DIRECTION('',(0.,0.,1.));
#11722=DIRECTION('center_axis',(0.,0.,-1.));
#11723=DIRECTION('ref_axis',(1.,0.,0.));
#11724=DIRECTION('center_axis',(0.,0.,1.));
#11725=DIRECTION('ref_axis',(1.,0.,0.));
#11726=DIRECTION('center_axis',(0.,0.,1.));
#11727=DIRECTION('ref_axis',(1.,0.,0.));
#11728=DIRECTION('',(0.,-1.,0.));
#11729=DIRECTION('center_axis',(0.,0.,1.));
#11730=DIRECTION('ref_axis',(1.,0.,0.));
#11731=DIRECTION('center_axis',(0.,0.,1.));
#11732=DIRECTION('ref_axis',(1.,0.,0.));
#11733=DIRECTION('',(0.,0.,1.));
#11734=DIRECTION('center_axis',(0.,0.,1.));
#11735=DIRECTION('ref_axis',(1.,0.,0.));
#11736=DIRECTION('',(0.,0.,-1.));
#11737=DIRECTION('center_axis',(0.,0.,1.));
#11738=DIRECTION('ref_axis',(-1.,1.22464679914735E-16,0.));
#11739=DIRECTION('',(0.,0.,-1.));
#11740=DIRECTION('center_axis',(0.,0.,1.));
#11741=DIRECTION('ref_axis',(1.,0.,0.));
#11742=DIRECTION('',(0.,0.,1.));
#11743=DIRECTION('center_axis',(0.,0.,1.));
#11744=DIRECTION('ref_axis',(1.,0.,0.));
#11745=DIRECTION('center_axis',(0.,0.,1.));
#11746=DIRECTION('ref_axis',(1.,0.,0.));
#11747=DIRECTION('',(0.,1.,0.));
#11748=DIRECTION('center_axis',(-1.,0.,0.));
#11749=DIRECTION('ref_axis',(0.,-1.,0.));
#11750=DIRECTION('',(0.,-1.,0.));
#11751=DIRECTION('',(0.,0.,1.));
#11752=DIRECTION('',(0.,-1.,0.));
#11753=DIRECTION('',(0.,0.,1.));
#11754=DIRECTION('',(0.,-1.,0.));
#11755=DIRECTION('center_axis',(0.,0.,1.));
#11756=DIRECTION('ref_axis',(1.,0.,0.));
#11757=DIRECTION('center_axis',(0.,0.,1.));
#11758=DIRECTION('ref_axis',(1.,0.,0.));
#11759=DIRECTION('',(0.,0.,1.));
#11760=DIRECTION('center_axis',(0.,0.,1.));
#11761=DIRECTION('ref_axis',(1.,0.,0.));
#11762=DIRECTION('center_axis',(0.,0.,1.));
#11763=DIRECTION('ref_axis',(1.,0.,0.));
#11764=DIRECTION('center_axis',(0.,0.,1.));
#11765=DIRECTION('ref_axis',(1.,0.,0.));
#11766=DIRECTION('center_axis',(0.,0.,1.));
#11767=DIRECTION('ref_axis',(1.,0.,0.));
#11768=DIRECTION('',(0.,0.,1.));
#11769=DIRECTION('center_axis',(0.,0.,1.));
#11770=DIRECTION('ref_axis',(1.,0.,0.));
#11771=DIRECTION('center_axis',(0.,0.,1.));
#11772=DIRECTION('ref_axis',(1.,0.,0.));
#11773=DIRECTION('center_axis',(0.,0.,1.));
#11774=DIRECTION('ref_axis',(1.,0.,0.));
#11775=DIRECTION('',(-1.,0.,0.));
#11776=DIRECTION('center_axis',(0.,0.,1.));
#11777=DIRECTION('ref_axis',(1.,0.,0.));
#11778=DIRECTION('center_axis',(0.,0.,1.));
#11779=DIRECTION('ref_axis',(1.,0.,0.));
#11780=DIRECTION('',(0.,0.,-1.));
#11781=DIRECTION('',(0.,0.,1.));
#11782=DIRECTION('center_axis',(0.,0.,-1.));
#11783=DIRECTION('ref_axis',(1.,0.,0.));
#11784=DIRECTION('',(0.,0.,1.));
#11785=DIRECTION('center_axis',(0.,1.,0.));
#11786=DIRECTION('ref_axis',(1.,0.,0.));
#11787=DIRECTION('center_axis',(0.,1.,0.));
#11788=DIRECTION('ref_axis',(1.,0.,0.));
#11789=DIRECTION('center_axis',(0.,1.,0.));
#11790=DIRECTION('ref_axis',(1.,0.,0.));
#11791=DIRECTION('center_axis',(0.,0.,1.));
#11792=DIRECTION('ref_axis',(1.,0.,0.));
#11793=DIRECTION('',(-1.,0.,0.));
#11794=DIRECTION('center_axis',(0.,0.,1.));
#11795=DIRECTION('ref_axis',(1.,0.,0.));
#11796=DIRECTION('center_axis',(0.,0.,1.));
#11797=DIRECTION('ref_axis',(6.12323399573677E-17,1.,0.));
#11798=DIRECTION('',(0.,0.,-1.));
#11799=DIRECTION('center_axis',(0.,0.,-1.));
#11800=DIRECTION('ref_axis',(1.,0.,0.));
#11801=DIRECTION('',(0.,0.,1.));
#11802=DIRECTION('center_axis',(0.,-1.,0.));
#11803=DIRECTION('ref_axis',(1.,0.,0.));
#11804=DIRECTION('',(1.,0.,0.));
#11805=DIRECTION('',(1.,0.,0.));
#11806=DIRECTION('',(0.,0.,1.));
#11807=DIRECTION('',(1.,0.,0.));
#11808=DIRECTION('center_axis',(0.,1.,0.));
#11809=DIRECTION('ref_axis',(1.,0.,0.));
#11810=DIRECTION('center_axis',(0.,1.,0.));
#11811=DIRECTION('ref_axis',(1.,0.,0.));
#11812=DIRECTION('center_axis',(0.,1.,0.));
#11813=DIRECTION('ref_axis',(1.,0.,0.));
#11814=DIRECTION('center_axis',(0.,1.,0.));
#11815=DIRECTION('ref_axis',(1.,0.,0.));
#11816=DIRECTION('center_axis',(0.,1.,0.));
#11817=DIRECTION('ref_axis',(1.,0.,0.));
#11818=DIRECTION('center_axis',(0.,1.,0.));
#11819=DIRECTION('ref_axis',(1.,0.,0.));
#11820=DIRECTION('',(0.,1.,0.));
#11821=DIRECTION('center_axis',(0.,-1.,0.));
#11822=DIRECTION('ref_axis',(1.,0.,0.));
#11823=DIRECTION('center_axis',(0.,1.,0.));
#11824=DIRECTION('ref_axis',(1.,0.,0.));
#11825=DIRECTION('',(0.,1.,0.));
#11826=DIRECTION('center_axis',(0.,-1.,0.));
#11827=DIRECTION('ref_axis',(1.,0.,0.));
#11828=DIRECTION('center_axis',(0.,1.,0.));
#11829=DIRECTION('ref_axis',(1.,0.,0.));
#11830=DIRECTION('',(0.,1.,0.));
#11831=DIRECTION('center_axis',(0.,-1.,0.));
#11832=DIRECTION('ref_axis',(1.,0.,0.));
#11833=DIRECTION('center_axis',(0.,1.,0.));
#11834=DIRECTION('ref_axis',(1.,0.,0.));
#11835=DIRECTION('',(0.,1.,0.));
#11836=DIRECTION('center_axis',(0.,-1.,0.));
#11837=DIRECTION('ref_axis',(1.,0.,0.));
#11838=DIRECTION('center_axis',(0.,1.,0.));
#11839=DIRECTION('ref_axis',(1.,0.,0.));
#11840=DIRECTION('',(0.,1.,0.));
#11841=DIRECTION('center_axis',(0.,1.,0.));
#11842=DIRECTION('ref_axis',(-1.,0.,0.));
#11843=DIRECTION('',(-1.,0.,0.));
#11844=DIRECTION('',(-1.,0.,0.));
#11845=DIRECTION('',(0.,0.,1.));
#11846=DIRECTION('center_axis',(1.,0.,0.));
#11847=DIRECTION('ref_axis',(0.,1.,0.));
#11848=DIRECTION('',(0.,1.,0.));
#11849=DIRECTION('',(0.,1.,0.));
#11850=DIRECTION('',(0.,1.,0.));
#11851=DIRECTION('center_axis',(0.,0.,1.));
#11852=DIRECTION('ref_axis',(1.,0.,0.));
#11853=DIRECTION('center_axis',(0.,0.,1.));
#11854=DIRECTION('ref_axis',(1.,0.,0.));
#14832=CARTESIAN_POINT('',(0.,0.,0.));
#14833=CARTESIAN_POINT('Origin',(-0.7,12.1,5.9));
#14834=CARTESIAN_POINT('',(-0.865,12.1,5.9));
#14835=CARTESIAN_POINT('Origin',(-0.7,12.1,5.9));
#14836=CARTESIAN_POINT('',(-0.865,12.1,7.));
#14837=CARTESIAN_POINT('',(-0.865,12.1,5.9));
#14838=CARTESIAN_POINT('Origin',(-0.7,12.1,7.));
#14839=CARTESIAN_POINT('Origin',(-0.7,12.1,5.9));
#14840=CARTESIAN_POINT('Origin',(0.7,12.1,5.9));
#14841=CARTESIAN_POINT('',(0.535,12.1,5.9));
#14842=CARTESIAN_POINT('Origin',(0.7,12.1,5.9));
#14843=CARTESIAN_POINT('',(0.535,12.1,7.));
#14844=CARTESIAN_POINT('',(0.535,12.1,5.9));
#14845=CARTESIAN_POINT('Origin',(0.7,12.1,7.));
#14846=CARTESIAN_POINT('Origin',(0.7,12.1,5.9));
#14847=CARTESIAN_POINT('Origin',(-2.9,11.7,2.6));
#14848=CARTESIAN_POINT('',(-2.5,12.0400367627184,2.6));
#14849=CARTESIAN_POINT('',(-2.5,11.3599632372816,2.6));
#14850=CARTESIAN_POINT('',(-2.5,12.15,2.6));
#14851=CARTESIAN_POINT('Origin',(-2.9,11.7,2.6));
#14852=CARTESIAN_POINT('Origin',(-2.9,11.7,2.));
#14853=CARTESIAN_POINT('',(-2.5,12.0400367627184,2.));
#14854=CARTESIAN_POINT('',(-2.5,12.0400367627184,2.));
#14855=CARTESIAN_POINT('',(-2.5,11.3599632372816,2.));
#14856=CARTESIAN_POINT('Origin',(-2.9,11.7,2.));
#14857=CARTESIAN_POINT('',(-2.5,11.3599632372816,2.));
#14858=CARTESIAN_POINT('Origin',(2.9,11.7,2.));
#14859=CARTESIAN_POINT('',(2.5,12.0400367627184,2.6));
#14860=CARTESIAN_POINT('',(2.5,12.0400367627184,2.));
#14861=CARTESIAN_POINT('',(2.5,12.0400367627184,2.));
#14862=CARTESIAN_POINT('',(2.5,11.3599632372816,2.6));
#14863=CARTESIAN_POINT('Origin',(2.9,11.7,2.6));
#14864=CARTESIAN_POINT('',(2.5,11.3599632372816,2.));
#14865=CARTESIAN_POINT('',(2.5,11.3599632372816,2.));
#14866=CARTESIAN_POINT('Origin',(2.9,11.7,2.));
#14867=CARTESIAN_POINT('Origin',(2.9,11.7,2.6));
#14868=CARTESIAN_POINT('',(2.5,11.3,2.6));
#14869=CARTESIAN_POINT('Origin',(-2.5,12.6,2.));
#14870=CARTESIAN_POINT('',(-2.5,10.9,2.));
#14871=CARTESIAN_POINT('',(-2.5,12.6,2.));
#14872=CARTESIAN_POINT('',(-2.5,10.9,7.));
#14873=CARTESIAN_POINT('',(-2.5,10.9,2.));
#14874=CARTESIAN_POINT('',(-2.5,12.6,7.));
#14875=CARTESIAN_POINT('',(-2.5,12.6,7.));
#14876=CARTESIAN_POINT('',(-2.5,12.6,2.));
#14877=CARTESIAN_POINT('',(-2.5,12.6,2.));
#14878=CARTESIAN_POINT('',(-2.5,12.6,2.));
#14879=CARTESIAN_POINT('Origin',(-1.2,12.,1.9));
#14880=CARTESIAN_POINT('',(-1.41,12.,2.));
#14881=CARTESIAN_POINT('Origin',(-1.2,12.,2.));
#14882=CARTESIAN_POINT('',(-1.41,12.,3.1));
#14883=CARTESIAN_POINT('',(-1.41,12.,1.9));
#14884=CARTESIAN_POINT('Origin',(-1.2,12.,3.1));
#14885=CARTESIAN_POINT('Origin',(-1.2,12.,3.1));
#14886=CARTESIAN_POINT('Origin',(1.2,12.,1.9));
#14887=CARTESIAN_POINT('',(0.99,12.,2.));
#14888=CARTESIAN_POINT('Origin',(1.2,12.,2.));
#14889=CARTESIAN_POINT('',(0.99,12.,3.1));
#14890=CARTESIAN_POINT('',(0.99,12.,1.9));
#14891=CARTESIAN_POINT('Origin',(1.2,12.,3.1));
#14892=CARTESIAN_POINT('Origin',(1.2,12.,3.1));
#14893=CARTESIAN_POINT('Origin',(0.,11.4,4.4));
#14894=CARTESIAN_POINT('',(0.2,11.4,4.4));
#14895=CARTESIAN_POINT('',(-0.2,11.4,4.4));
#14896=CARTESIAN_POINT('',(0.,11.4,4.4));
#14897=CARTESIAN_POINT('Origin',(0.,11.4,4.4));
#14898=CARTESIAN_POINT('Origin',(0.,11.4,4.4));
#14899=CARTESIAN_POINT('',(0.2,11.4,5.73389626792531));
#14900=CARTESIAN_POINT('',(0.2,11.4,4.4));
#14901=CARTESIAN_POINT('',(-0.2,11.4,5.73389626792531));
#14902=CARTESIAN_POINT('Ctrl Pts',(-0.2,11.4,5.73389626792531));
#14903=CARTESIAN_POINT('Ctrl Pts',(-0.2,11.3748407538878,5.73389626792531));
#14904=CARTESIAN_POINT('Ctrl Pts',(-0.194963049432274,11.3480346466781,
5.73474532770021));
#14905=CARTESIAN_POINT('Ctrl Pts',(-0.1745390117426,11.2987719239996,5.73779753882153));
#14906=CARTESIAN_POINT('Ctrl Pts',(-0.159154241644127,11.2763115291695,
5.73995502329995));
#14907=CARTESIAN_POINT('Ctrl Pts',(-0.123688872270436,11.2408461597958,
5.74399340066366));
#14908=CARTESIAN_POINT('Ctrl Pts',(-0.101228304743543,11.2254610747931,
5.7461387706165));
#14909=CARTESIAN_POINT('Ctrl Pts',(-0.0519649901302408,11.2050368082905,
5.74916317792714));
#14910=CARTESIAN_POINT('Ctrl Pts',(-0.0251586765531237,11.2,5.75));
#14911=CARTESIAN_POINT('Ctrl Pts',(0.0251586765531237,11.2,5.75));
#14912=CARTESIAN_POINT('Ctrl Pts',(0.0519649901302413,11.2050368082905,
5.74916317792714));
#14913=CARTESIAN_POINT('Ctrl Pts',(0.101228304743543,11.2254610747931,5.7461387706165));
#14914=CARTESIAN_POINT('Ctrl Pts',(0.123688872270436,11.2408461597958,5.74399340066366));
#14915=CARTESIAN_POINT('Ctrl Pts',(0.159154241644127,11.2763115291695,5.73995502329995));
#14916=CARTESIAN_POINT('Ctrl Pts',(0.1745390117426,11.2987719239996,5.73779753882153));
#14917=CARTESIAN_POINT('Ctrl Pts',(0.194963049432274,11.3480346466781,5.73474532770021));
#14918=CARTESIAN_POINT('Ctrl Pts',(0.2,11.3748407538878,5.73389626792531));
#14919=CARTESIAN_POINT('Ctrl Pts',(0.2,11.4,5.73389626792531));
#14920=CARTESIAN_POINT('',(-0.2,11.4,6.35));
#14921=CARTESIAN_POINT('',(-0.2,11.4,4.4));
#14922=CARTESIAN_POINT('Origin',(0.,11.4,6.35));
#14923=CARTESIAN_POINT('',(-0.2,11.4,4.4));
#14924=CARTESIAN_POINT('Origin',(0.,11.4,4.5));
#14925=CARTESIAN_POINT('',(-1.25,11.4,4.5));
#14926=CARTESIAN_POINT('Origin',(0.,11.4,4.5));
#14927=CARTESIAN_POINT('Origin',(0.,11.4,4.5));
#14928=CARTESIAN_POINT('Origin',(0.,11.4,6.35));
#14929=CARTESIAN_POINT('',(0.123389626792531,10.9,6.35));
#14930=CARTESIAN_POINT('',(-0.123389626792531,10.9,6.35));
#14931=CARTESIAN_POINT('',(-1.25,10.9,6.35));
#14932=CARTESIAN_POINT('Origin',(0.,11.4,6.35));
#14933=CARTESIAN_POINT('Origin',(0.,11.4,6.35));
#14934=CARTESIAN_POINT('',(0.123389626792531,10.9,7.));
#14935=CARTESIAN_POINT('',(0.123389626792531,10.9,6.35));
#14936=CARTESIAN_POINT('',(-0.123389626792531,10.9,7.));
#14937=CARTESIAN_POINT('Origin',(0.,11.4,7.));
#14938=CARTESIAN_POINT('',(-0.123389626792531,10.9,6.35));
#14939=CARTESIAN_POINT('Origin',(-2.5,10.9,2.));
#14940=CARTESIAN_POINT('',(-2.5,10.9,7.));
#14941=CARTESIAN_POINT('',(2.5,10.9,2.));
#14942=CARTESIAN_POINT('',(-2.5,10.9,2.));
#14943=CARTESIAN_POINT('',(2.5,10.9,7.));
#14944=CARTESIAN_POINT('',(2.5,10.9,2.));
#14945=CARTESIAN_POINT('',(-2.5,10.9,7.));
#14946=CARTESIAN_POINT('',(1.725,10.9,2.5));
#14947=CARTESIAN_POINT('Origin',(2.,10.9,2.5));
#14948=CARTESIAN_POINT('',(-2.275,10.9,6.5));
#14949=CARTESIAN_POINT('Origin',(-2.,10.9,6.5));
#14950=CARTESIAN_POINT('',(-2.275,10.9,2.5));
#14951=CARTESIAN_POINT('Origin',(-2.,10.9,2.5));
#14952=CARTESIAN_POINT('',(1.725,10.9,6.5));
#14953=CARTESIAN_POINT('Origin',(2.,10.9,6.5));
#14954=CARTESIAN_POINT('',(-1.25,10.9,4.5));
#14955=CARTESIAN_POINT('Origin',(0.,10.9,4.5));
#14956=CARTESIAN_POINT('Origin',(2.,10.8,2.5));
#14957=CARTESIAN_POINT('',(1.725,12.6,2.5));
#14958=CARTESIAN_POINT('',(1.725,10.8,2.5));
#14959=CARTESIAN_POINT('Origin',(2.,12.6,2.5));
#14960=CARTESIAN_POINT('Origin',(-2.,10.8,6.5));
#14961=CARTESIAN_POINT('',(-2.275,12.6,6.5));
#14962=CARTESIAN_POINT('',(-2.275,10.8,6.5));
#14963=CARTESIAN_POINT('Origin',(-2.,12.6,6.5));
#14964=CARTESIAN_POINT('Origin',(-2.,10.8,2.5));
#14965=CARTESIAN_POINT('',(-2.275,12.6,2.5));
#14966=CARTESIAN_POINT('',(-2.275,10.8,2.5));
#14967=CARTESIAN_POINT('Origin',(-2.,12.6,2.5));
#14968=CARTESIAN_POINT('Origin',(2.,10.8,6.5));
#14969=CARTESIAN_POINT('',(1.725,12.6,6.5));
#14970=CARTESIAN_POINT('',(1.725,10.8,6.5));
#14971=CARTESIAN_POINT('Origin',(2.,12.6,6.5));
#14972=CARTESIAN_POINT('Origin',(0.,10.8,4.5));
#14973=CARTESIAN_POINT('',(-1.25,10.8,4.5));
#14974=CARTESIAN_POINT('Origin',(2.5,12.6,2.));
#14975=CARTESIAN_POINT('',(2.5,12.6,2.));
#14976=CARTESIAN_POINT('',(2.5,12.6,2.));
#14977=CARTESIAN_POINT('',(2.5,12.6,7.));
#14978=CARTESIAN_POINT('',(2.5,12.6,7.));
#14979=CARTESIAN_POINT('',(2.5,12.6,2.));
#14980=CARTESIAN_POINT('Origin',(2.5,10.9,2.));
#14981=CARTESIAN_POINT('',(2.5,10.9,2.));
#14982=CARTESIAN_POINT('',(2.5,10.9,7.));
#14983=CARTESIAN_POINT('',(2.5,10.9,2.));
#14984=CARTESIAN_POINT('Origin',(0.,11.75,7.));
#14985=CARTESIAN_POINT('Origin',(0.,11.75,2.));
#18906=UNCERTAINTY_MEASURE_WITH_UNIT(LENGTH_MEASURE(0.001),#19044,
'DISTANCE_ACCURACY_VALUE',
'Maximum model space distance between geometric entities at asserted c
onnectivities');
#18972=UNCERTAINTY_MEASURE_WITH_UNIT(LENGTH_MEASURE(0.001),#19044,
'DISTANCE_ACCURACY_VALUE',
'Maximum model space distance between geometric entities at asserted c
onnectivities');
#18977=(
GEOMETRIC_REPRESENTATION_CONTEXT(3)
GLOBAL_UNCERTAINTY_ASSIGNED_CONTEXT((#18906))
GLOBAL_UNIT_ASSIGNED_CONTEXT((#19044,#19046,#19047))
REPRESENTATION_CONTEXT('','3D')
);
#19043=(
GEOMETRIC_REPRESENTATION_CONTEXT(3)
GLOBAL_UNCERTAINTY_ASSIGNED_CONTEXT((#18972))
GLOBAL_UNIT_ASSIGNED_CONTEXT((#19044,#19046,#19047))
REPRESENTATION_CONTEXT('','3D')
);
#19044=(
LENGTH_UNIT()
NAMED_UNIT(*)
SI_UNIT(.CENTI.,.METRE.)
);
#19046=(
NAMED_UNIT(*)
PLANE_ANGLE_UNIT()
SI_UNIT($,.RADIAN.)
);
#19047=(
NAMED_UNIT(*)
SI_UNIT($,.STERADIAN.)
SOLID_ANGLE_UNIT()
);
#19052=SHAPE_DEFINITION_REPRESENTATION(#19122,#19310);
#19122=PRODUCT_DEFINITION_SHAPE('',$,#19381);
#19310=SHAPE_REPRESENTATION('',(#10322),#18977);
#19376=PRODUCT_DEFINITION_CONTEXT('part definition',#19588,'design');
#19381=PRODUCT_DEFINITION('2026-11-03-00-38-46-438','Rear cap',#19451,#19376);
#19451=PRODUCT_DEFINITION_FORMATION('',$,#19594);
#19588=APPLICATION_CONTEXT(
'Core Data for Automotive Mechanical Design Process');
#19589=PRODUCT_CONTEXT('part definition',#19588,'mechanical');
#19594=PRODUCT('2026-11-03-00-38-46-438','Rear cap','Rear cap',(#19589));
#19661=PRESENTATION_STYLE_ASSIGNMENT((#19667));
#19667=SURFACE_STYLE_USAGE(.BOTH.,#19673);
#19673=SURFACE_SIDE_STYLE('',(#19679));
#19679=SURFACE_STYLE_FILL_AREA(#19685);
#19685=FILL_AREA_STYLE('CAD Library Painted - Engineering blue',(#19691));
#19691=FILL_AREA_STYLE_COLOUR('CAD Library Painted - Engineering blue',
#19697);
#19697=COLOUR_RGB('CAD Library Painted - Engineering blue',0.12156862745098,
0.356862745098039,0.6);
ENDSEC;
END-ISO-10303-21;
